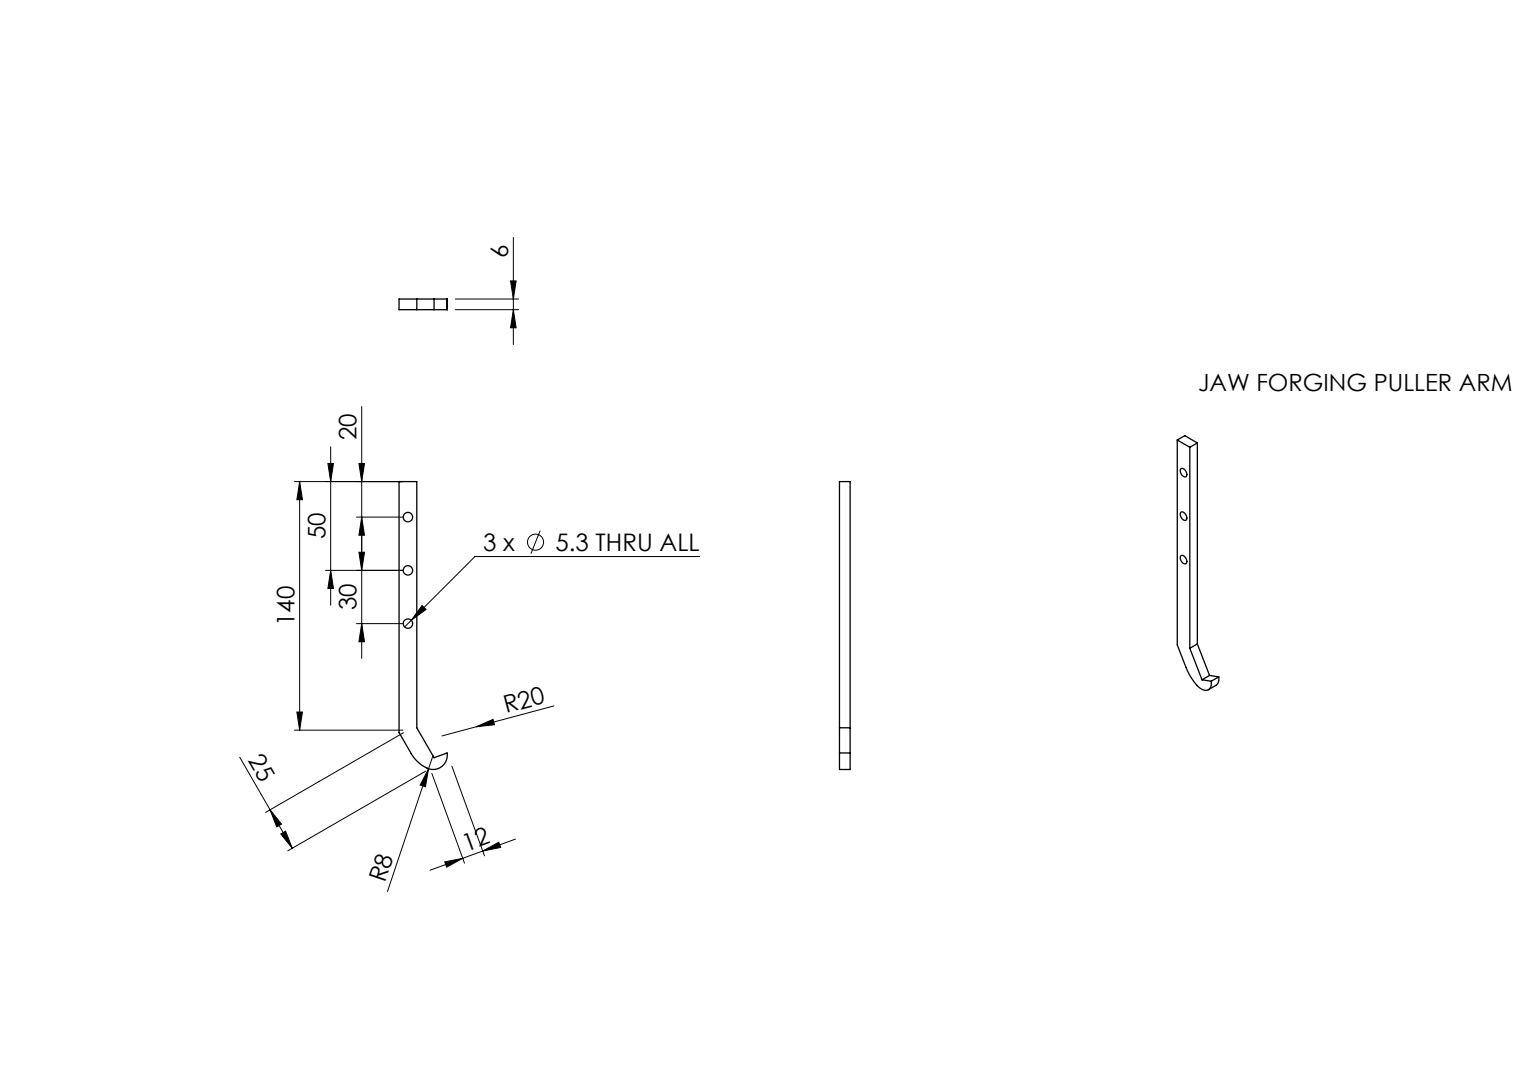
ISO-10303-21;
HEADER;
FILE_DESCRIPTION (('STEP AP214'),
    '1' );
FILE_NAME ('Jaw Forging Puller Arm.step',
    '2026-10-22T13:24:12',
    ( '' ),
    ( '' ),
    'SwSTEP 2.0',
    'SolidWorks 2026',
    '' );
FILE_SCHEMA (( 'AUTOMOTIVE_DESIGN' ));
ENDSEC;

DATA;
#1=DIRECTION ( 'NONE',  ( 1.000000000000000000, 0.000000000000000000, 0.000000000000000000 ) ) ;
#20=PRODUCT_DEFINITION_SHAPE ( 'NONE', 'NONE',  #1387 ) ;
#22=VECTOR ( 'NONE', #2319, 1000.000000000000000 ) ;
#55=EDGE_CURVE ( 'NONE', #2070, #608, #62, .T. ) ;
#59=CARTESIAN_POINT ( 'NONE',  ( -58.09974666316955449, -143.2580143298517328, -3.000000000000000000 ) ) ;
#62=CIRCLE ( 'NONE', #204, 20.00000000000000355 ) ;
#63=AXIS2_PLACEMENT_3D ( 'NONE', #554, #2133, #1693 ) ;
#75=EDGE_CURVE ( 'NONE', #120, #1771, #154, .T. ) ;
#76=CYLINDRICAL_SURFACE ( 'NONE', #302, 2.649999999999985700 ) ;
#78=LINE ( 'NONE', #2340, #2456 ) ;
#83=VERTEX_POINT ( 'NONE', #98 ) ;
#91=DIRECTION ( 'NONE',  ( -0.000000000000000000, -0.000000000000000000, 1.000000000000000000 ) ) ;
#93=VERTEX_POINT ( 'NONE', #2360 ) ;
#94=AXIS2_PLACEMENT_3D ( 'NONE', #273, #1403, #2068 ) ;
#98=CARTESIAN_POINT ( 'NONE',  ( -62.63076211353318712, -9.999999999999943157, 3.000000000000001332 ) ) ;
#109=CLOSED_SHELL ( 'NONE', ( #2797, #1837, #1415, #550, #392, #827, #441, #1532, #2192, #615, #2313, #2289, #2566, #2325, #660, #1443, #890 ) ) ;
#111=EDGE_CURVE ( 'NONE', #2201, #2834, #2628, .T. ) ;
#113=EDGE_CURVE ( 'NONE', #132, #2201, #803, .T. ) ;
#120=VERTEX_POINT ( 'NONE', #127 ) ;
#125=ORIENTED_EDGE ( 'NONE', *, *, #2038, .F. ) ;
#127=CARTESIAN_POINT ( 'NONE',  ( -37.91455138073065001, -142.8479302707733041, -3.000000000000000000 ) ) ;
#128=CARTESIAN_POINT ( 'NONE',  ( -62.63076211353317291, -39.99999999999994316, -3.000000000000005329 ) ) ;
#129=EDGE_CURVE ( 'NONE', #732, #608, #1011, .T. ) ;
#131=DIRECTION ( 'NONE',  ( -0.000000000000000000, -0.000000000000000000, 1.000000000000000000 ) ) ;
#132=VERTEX_POINT ( 'NONE', #1872 ) ;
#134=( NAMED_UNIT ( * ) PLANE_ANGLE_UNIT ( ) SI_UNIT ( $, .RADIAN. ) );
#143=CARTESIAN_POINT ( 'NONE',  ( -57.33076211353320417, -69.99999999999995737, 3.000000000000001332 ) ) ;
#152=EDGE_CURVE ( 'NONE', #1771, #732, #1431, .T. ) ;
#154=CIRCLE ( 'NONE', #1792, 8.000000000000000000 ) ;
#160=DIRECTION ( 'NONE',  ( 1.000000000000000000, 0.000000000000000000, 0.000000000000000000 ) ) ;
#167=VERTEX_POINT ( 'NONE', #2852 ) ;
#171=ORIENTED_EDGE ( 'NONE', *, *, #2056, .F. ) ;
#175=DIRECTION ( 'NONE',  ( 1.000000000000000000, 0.000000000000000000, 0.000000000000000000 ) ) ;
#177=ORIENTED_EDGE ( 'NONE', *, *, #2792, .T. ) ;
#190=LINE ( 'NONE', #904, #997 ) ;
#197=VECTOR ( 'NONE', #522, 1000.000000000000000 ) ;
#199=EDGE_CURVE ( 'NONE', #2240, #2529, #1039, .T. ) ;
#204=AXIS2_PLACEMENT_3D ( 'NONE', #900, #2724, #531 ) ;
#211=CARTESIAN_POINT ( 'NONE',  ( -59.98076211353318854, -69.99999999999995737, 3.000000000000000000 ) ) ;
#212=VECTOR ( 'NONE', #1969, 1000.000000000000000 ) ;
#214=LINE ( 'NONE', #690, #2553 ) ;
#219=EDGE_CURVE ( 'NONE', #1447, #1073, #1678, .T. ) ;
#223=DIRECTION ( 'NONE',  ( -1.000000000000000000, 0.000000000000000000, 0.000000000000000000 ) ) ;
#224=CARTESIAN_POINT ( 'NONE',  ( -59.98076211353319565, -9.999999999999943157, 3.000000000000000000 ) ) ;
#230=CARTESIAN_POINT ( 'NONE',  ( -64.98076211353318854, 10.00000000000005684, -3.000000000000000000 ) ) ;
#231=CARTESIAN_POINT ( 'NONE',  ( 0.000000000000000000, 0.000000000000000000, 0.000000000000000000 ) ) ;
#232=ORIENTED_EDGE ( 'NONE', *, *, #2574, .F. ) ;
#233=EDGE_CURVE ( 'NONE', #1447, #2315, #1733, .T. ) ;
#245=DIRECTION ( 'NONE',  ( 0.000000000000000000, 0.000000000000000000, 1.000000000000000000 ) ) ;
#247=ORIENTED_EDGE ( 'NONE', *, *, #2110, .T. ) ;
#249=CARTESIAN_POINT ( 'NONE',  ( -37.80724301738815285, -144.1538470861320604, -3.000000000000000000 ) ) ;
#252=CARTESIAN_POINT ( 'NONE',  ( -40.77923858748079766, -133.2580143298517044, -3.000000000000000000 ) ) ;
#254=VECTOR ( 'NONE', #2412, 1000.000000000000000 ) ;
#257=EDGE_CURVE ( 'NONE', #2834, #1447, #2641, .T. ) ;
#263=SURFACE_STYLE_USAGE ( .BOTH. , #928 ) ;
#266=( NAMED_UNIT ( * ) PLANE_ANGLE_UNIT ( ) SI_UNIT ( $, .RADIAN. ) );
#270=CARTESIAN_POINT ( 'NONE',  ( -49.19086283016151384, -146.9521719906813928, 3.000000000000000000 ) ) ;
#273=CARTESIAN_POINT ( 'NONE',  ( 0.000000000000000000, 0.000000000000000000, -3.000000000000000000 ) ) ;
#274=ORIENTED_EDGE ( 'NONE', *, *, #2038, .T. ) ;
#277=ORIENTED_EDGE ( 'NONE', *, *, #2792, .F. ) ;
#281=CARTESIAN_POINT ( 'NONE',  ( -59.98076211353318854, -69.99999999999995737, -3.000000000000005329 ) ) ;
#282=EDGE_CURVE ( 'NONE', #300, #2070, #409, .T. ) ;
#289=ORIENTED_EDGE ( 'NONE', *, *, #762, .F. ) ;
#295=VECTOR ( 'NONE', #821, 1000.000000000000000 ) ;
#300=VERTEX_POINT ( 'NONE', #2011 ) ;
#302=AXIS2_PLACEMENT_3D ( 'NONE', #1642, #1876, #2515 ) ;
#305=EDGE_LOOP ( 'NONE', ( #581, #1424, #2061, #2597 ) ) ;
#308=CARTESIAN_POINT ( 'NONE',  ( -55.65063509461099045, -127.4999999999999432, 3.000000000000000000 ) ) ;
#311=CARTESIAN_POINT ( 'NONE',  ( -62.63076211353317291, -69.99999999999995737, 3.000000000000000000 ) ) ;
#322=DIRECTION ( 'NONE',  ( 0.000000000000000000, -0.000000000000000000, 1.000000000000000000 ) ) ;
#333=CARTESIAN_POINT ( 'NONE',  ( -59.98076211353318854, -69.99999999999995737, 3.000000000000001332 ) ) ;
#334=ORIENTED_EDGE ( 'NONE', *, *, #1164, .F. ) ;
#336=AXIS2_PLACEMENT_3D ( 'NONE', #211, #2698, #2453 ) ;
#352=DIRECTION ( 'NONE',  ( 0.8660254037844379305, 0.5000000000000014433, -0.000000000000000000 ) ) ;
#356=DIRECTION ( 'NONE',  ( 1.000000000000000000, 0.000000000000000000, 0.000000000000000000 ) ) ;
#374=VECTOR ( 'NONE', #2202, 1000.000000000000000 ) ;
#378=ORIENTED_EDGE ( 'NONE', *, *, #113, .F. ) ;
#379=DIRECTION ( 'NONE',  ( -0.000000000000000000, -0.000000000000000000, 1.000000000000000000 ) ) ;
#384=CARTESIAN_POINT ( 'NONE',  ( -62.63076211353317291, -69.99999999999995737, 3.000000000000001332 ) ) ;
#387=CARTESIAN_POINT ( 'NONE',  ( -59.98076211353318854, -69.99999999999995737, 3.000000000000001332 ) ) ;
#388=VECTOR ( 'NONE', #1937, 1000.000000000000000 ) ;
#390=CARTESIAN_POINT ( 'NONE',  ( -54.98076211353318143, -128.6602540378443393, 3.000000000000000000 ) ) ;
#392=ADVANCED_FACE ( 'NONE', ( #2249 ), #1339, .T. ) ;
#401=CARTESIAN_POINT ( 'NONE',  ( -57.33076211353320417, -39.99999999999994316, -3.000000000000005329 ) ) ;
#409=LINE ( 'NONE', #626, #254 ) ;
#413=DIRECTION ( 'NONE',  ( -0.000000000000000000, -0.000000000000000000, 1.000000000000000000 ) ) ;
#416=AXIS2_PLACEMENT_3D ( 'NONE', #1762, #636, #1319 ) ;
#417=CARTESIAN_POINT ( 'NONE',  ( -45.80724301738815285, -144.1538470861320604, 3.000000000000000000 ) ) ;
#419=VECTOR ( 'NONE', #558, 1000.000000000000000 ) ;
#432=EDGE_LOOP ( 'NONE', ( #247, #171, #2273, #2867 ) ) ;
#434=CIRCLE ( 'NONE', #2909, 8.000000000000000000 ) ;
#436=VECTOR ( 'NONE', #2543, 1000.000000000000000 ) ;
#440=DIRECTION ( 'NONE',  ( -0.000000000000000000, -0.000000000000000000, 1.000000000000000000 ) ) ;
#441=ADVANCED_FACE ( 'NONE', ( #2720 ), #2522, .T. ) ;
#454=ORIENTED_EDGE ( 'NONE', *, *, #762, .T. ) ;
#466=COLOUR_RGB ( '',0.8941176470588234615, 0.8941176470588234615, 0.8941176470588234615 ) ;
#469=VECTOR ( 'NONE', #91, 1000.000000000000000 ) ;
#473=CYLINDRICAL_SURFACE ( 'NONE', #1427, 2.649999999999985700 ) ;
#478=UNCERTAINTY_MEASURE_WITH_UNIT (LENGTH_MEASURE( 1.000000000000000082E-05 ), #1953, 'distance_accuracy_value', 'NONE');
#487=ORIENTED_EDGE ( 'NONE', *, *, #685, .T. ) ;
#489=DIRECTION ( 'NONE',  ( -0.000000000000000000, -0.000000000000000000, 1.000000000000000000 ) ) ;
#495=EDGE_CURVE ( 'NONE', #1073, #120, #1819, .T. ) ;
#501=CARTESIAN_POINT ( 'NONE',  ( -62.63076211353318712, -9.999999999999943157, 3.000000000000000000 ) ) ;
#503=CARTESIAN_POINT ( 'NONE',  ( -57.33076211353320417, -69.99999999999995737, -3.000000000000005329 ) ) ;
#506=CARTESIAN_POINT ( 'NONE',  ( -62.63076211353317291, -39.99999999999994316, 3.000000000000000000 ) ) ;
#510=AXIS2_PLACEMENT_3D ( 'NONE', #2538, #1421, #1142 ) ;
#511=CARTESIAN_POINT ( 'NONE',  ( 0.000000000000000000, 0.000000000000000000, 3.000000000000000000 ) ) ;
#514=EDGE_CURVE ( 'NONE', #1931, #1630, #755, .T. ) ;
#522=DIRECTION ( 'NONE',  ( -0.000000000000000000, -0.000000000000000000, 1.000000000000000000 ) ) ;
#531=DIRECTION ( 'NONE',  ( -1.000000000000000000, 0.000000000000000000, 0.000000000000000000 ) ) ;
#536=CARTESIAN_POINT ( 'NONE',  ( -64.98076211353318854, 10.00000000000005684, 3.000000000000000000 ) ) ;
#546=DIRECTION ( 'NONE',  ( -0.000000000000000000, -0.000000000000000000, 1.000000000000000000 ) ) ;
#550=ADVANCED_FACE ( 'NONE', ( #589 ), #2548, .T. ) ;
#554=CARTESIAN_POINT ( 'NONE',  ( -45.80724301738815285, -144.1538470861320604, -3.000000000000000000 ) ) ;
#557=AXIS2_PLACEMENT_3D ( 'NONE', #1093, #1120, #664 ) ;
#558=DIRECTION ( 'NONE',  ( -0.000000000000000000, -0.000000000000000000, 1.000000000000000000 ) ) ;
#560=ORIENTED_EDGE ( 'NONE', *, *, #1193, .F. ) ;
#561=PLANE ( 'NONE',  #1135 ) ;
#563=ORIENTED_EDGE ( 'NONE', *, *, #2156, .F. ) ;
#564=AXIS2_PLACEMENT_3D ( 'NONE', #270, #2042, #727 ) ;
#575=ORIENTED_EDGE ( 'NONE', *, *, #2314, .T. ) ;
#578=EDGE_LOOP ( 'NONE', ( #232, #588 ) ) ;
#581=ORIENTED_EDGE ( 'NONE', *, *, #782, .F. ) ;
#583=EDGE_CURVE ( 'NONE', #1771, #167, #812, .T. ) ;
#586=LINE ( 'NONE', #1489, #295 ) ;
#588=ORIENTED_EDGE ( 'NONE', *, *, #1702, .F. ) ;
#589=FACE_OUTER_BOUND ( 'NONE', #1154, .T. ) ;
#591=CARTESIAN_POINT ( 'NONE',  ( -40.77923858748079766, -133.2580143298517044, 3.000000000000000000 ) ) ;
#606=EDGE_LOOP ( 'NONE', ( #2745, #2300, #1536, #1449, #625, #2303, #454, #2564, #695 ) ) ;
#608=VERTEX_POINT ( 'NONE', #2604 ) ;
#615=ADVANCED_FACE ( 'NONE', ( #1270 ), #561, .F. ) ;
#623=DIRECTION ( 'NONE',  ( -1.000000000000000000, 0.000000000000000000, 0.000000000000000000 ) ) ;
#625=ORIENTED_EDGE ( 'NONE', *, *, #1622, .F. ) ;
#626=CARTESIAN_POINT ( 'NONE',  ( -64.31088913245535821, -132.4999999999999432, 3.000000000000000000 ) ) ;
#634=EDGE_CURVE ( 'NONE', #2529, #2240, #2044, .T. ) ;
#636=DIRECTION ( 'NONE',  ( -0.000000000000000000, -0.000000000000000000, 1.000000000000000000 ) ) ;
#645=DIRECTION ( 'NONE',  ( -0.000000000000000000, -0.000000000000000000, 1.000000000000000000 ) ) ;
#653=ORIENTED_EDGE ( 'NONE', *, *, #752, .F. ) ;
#660=ADVANCED_FACE ( 'NONE', ( #798 ), #1966, .F. ) ;
#664=DIRECTION ( 'NONE',  ( -1.000000000000000000, 3.469446951953614189E-15, 0.000000000000000000 ) ) ;
#682=FACE_OUTER_BOUND ( 'NONE', #606, .T. ) ;
#685=EDGE_CURVE ( 'NONE', #167, #1073, #434, .T. ) ;
#688=CARTESIAN_POINT ( 'NONE',  ( -64.98076211353318854, 10.00000000000005684, 3.000000000000000000 ) ) ;
#690=CARTESIAN_POINT ( 'NONE',  ( -49.19086283016151384, -146.9521719906813928, -3.000000000000000000 ) ) ;
#695=ORIENTED_EDGE ( 'NONE', *, *, #1164, .T. ) ;
#707=PLANE ( 'NONE',  #2476 ) ;
#712=CIRCLE ( 'NONE', #1563, 2.649999999999985700 ) ;
#716=FACE_BOUND ( 'NONE', #813, .T. ) ;
#717=EDGE_LOOP ( 'NONE', ( #289, #2875, #2214, #2681 ) ) ;
#719=FACE_OUTER_BOUND ( 'NONE', #1079, .T. ) ;
#721=LINE ( 'NONE', #688, #436 ) ;
#722=FACE_OUTER_BOUND ( 'NONE', #717, .T. ) ;
#727=DIRECTION ( 'NONE',  ( -0.9396926207859063185, -0.3420201433256743195, 0.000000000000000000 ) ) ;
#728=FACE_BOUND ( 'NONE', #2290, .T. ) ;
#732=VERTEX_POINT ( 'NONE', #2497 ) ;
#736=VECTOR ( 'NONE', #1465, 1000.000000000000000 ) ;
#741=VERTEX_POINT ( 'NONE', #1537 ) ;
#742=DIRECTION ( 'NONE',  ( 1.000000000000000000, 0.000000000000000000, 0.000000000000000000 ) ) ;
#748=CARTESIAN_POINT ( 'NONE',  ( -62.63076211353317291, -69.99999999999995737, -3.000000000000005329 ) ) ;
#752=EDGE_CURVE ( 'NONE', #2529, #1384, #190, .T. ) ;
#755=CIRCLE ( 'NONE', #2422, 2.649999999999985700 ) ;
#760=DIRECTION ( 'NONE',  ( -1.000000000000000000, 0.000000000000000000, 0.000000000000000000 ) ) ;
#762=EDGE_CURVE ( 'NONE', #1742, #1508, #2230, .T. ) ;
#767=ORIENTED_EDGE ( 'NONE', *, *, #75, .F. ) ;
#770=DIRECTION ( 'NONE',  ( -0.000000000000000000, -0.000000000000000000, 1.000000000000000000 ) ) ;
#777=CARTESIAN_POINT ( 'NONE',  ( -37.80724301738815285, -144.1538470861320604, 3.000000000000000000 ) ) ;
#782=EDGE_CURVE ( 'NONE', #814, #969, #712, .T. ) ;
#788=CIRCLE ( 'NONE', #1596, 2.649999999999985700 ) ;
#792=AXIS2_PLACEMENT_3D ( 'NONE', #224, #2741, #1523 ) ;
#794=FACE_OUTER_BOUND ( 'NONE', #1190, .T. ) ;
#795=STYLED_ITEM('',(#2956),#1538);
#797=ORIENTED_EDGE ( 'NONE', *, *, #583, .F. ) ;
#798=FACE_OUTER_BOUND ( 'NONE', #1917, .T. ) ;
#800=ORIENTED_EDGE ( 'NONE', *, *, #1284, .T. ) ;
#803=LINE ( 'NONE', #1707, #1373 ) ;
#812=LINE ( 'NONE', #777, #2141 ) ;
#813=EDGE_LOOP ( 'NONE', ( #800, #1999 ) ) ;
#814=VERTEX_POINT ( 'NONE', #748 ) ;
#821=DIRECTION ( 'NONE',  ( 0.5000000000000013323, -0.8660254037844379305, 0.000000000000000000 ) ) ;
#827=ADVANCED_FACE ( 'NONE', ( #2062 ), #707, .T. ) ;
#832=ORIENTED_EDGE ( 'NONE', *, *, #872, .F. ) ;
#837=ORIENTED_EDGE ( 'NONE', *, *, #199, .T. ) ;
#843=CARTESIAN_POINT ( 'NONE',  ( -62.63076211353317291, -39.99999999999994316, 3.000000000000001332 ) ) ;
#844=ORIENTED_EDGE ( 'NONE', *, *, #514, .T. ) ;
#851=AXIS2_PLACEMENT_3D ( 'NONE', #1018, #379, #1728 ) ;
#854=VECTOR ( 'NONE', #546, 1000.000000000000000 ) ;
#857=LINE ( 'NONE', #1534, #1783 ) ;
#858=ORIENTED_EDGE ( 'NONE', *, *, #1284, .F. ) ;
#860=CYLINDRICAL_SURFACE ( 'NONE', #336, 2.649999999999985700 ) ;
#866=SHAPE_DEFINITION_REPRESENTATION ( #20, #1396 ) ;
#872=EDGE_CURVE ( 'NONE', #2834, #93, #916, .T. ) ;
#887=PRODUCT_DEFINITION_CONTEXT ( 'detailed design', #2350, 'design' ) ;
#890=ADVANCED_FACE ( 'NONE', ( #2291 ), #76, .F. ) ;
#900=CARTESIAN_POINT ( 'NONE',  ( -40.77923858748079766, -133.2580143298517044, 3.000000000000000000 ) ) ;
#904=CARTESIAN_POINT ( 'NONE',  ( -57.33076211353321128, -9.999999999999943157, 3.000000000000000000 ) ) ;
#908=VERTEX_POINT ( 'NONE', #59 ) ;
#909=DIRECTION ( 'NONE',  ( 1.000000000000000000, 1.486905836551548586E-16, -0.000000000000000000 ) ) ;
#916=LINE ( 'NONE', #1395, #22 ) ;
#921=ORIENTED_EDGE ( 'NONE', *, *, #1009, .T. ) ;
#928=SURFACE_SIDE_STYLE ('',( #1344 ) ) ;
#941=AXIS2_PLACEMENT_3D ( 'NONE', #536, #2097, #322 ) ;
#944=CARTESIAN_POINT ( 'NONE',  ( -59.98076211353319565, -9.999999999999943157, 3.000000000000000000 ) ) ;
#954=ORIENTED_EDGE ( 'NONE', *, *, #2516, .F. ) ;
#956=FACE_OUTER_BOUND ( 'NONE', #2363, .T. ) ;
#959=DIRECTION ( 'NONE',  ( -0.000000000000000000, -0.000000000000000000, 1.000000000000000000 ) ) ;
#962=LINE ( 'NONE', #1832, #2751 ) ;
#964=EDGE_CURVE ( 'NONE', #132, #300, #721, .T. ) ;
#968=DIRECTION ( 'NONE',  ( 0.000000000000000000, 0.000000000000000000, -1.000000000000000000 ) ) ;
#969=VERTEX_POINT ( 'NONE', #503 ) ;
#986=( GEOMETRIC_REPRESENTATION_CONTEXT ( 3 ) GLOBAL_UNCERTAINTY_ASSIGNED_CONTEXT ( ( #478 ) ) GLOBAL_UNIT_ASSIGNED_CONTEXT ( ( #1953, #134, #1510 ) ) REPRESENTATION_CONTEXT ( 'NONE', 'WORKASPACE' ) );
#995=ORIENTED_EDGE ( 'NONE', *, *, #583, .T. ) ;
#997=VECTOR ( 'NONE', #2713, 1000.000000000000000 ) ;
#1009=EDGE_CURVE ( 'NONE', #969, #1547, #2586, .T. ) ;
#1011=LINE ( 'NONE', #1668, #2903 ) ;
#1013=CARTESIAN_POINT ( 'NONE',  ( -64.98076211353316012, -131.3397459621555754, 3.000000000000000000 ) ) ;
#1014=ORIENTED_EDGE ( 'NONE', *, *, #634, .T. ) ;
#1018=CARTESIAN_POINT ( 'NONE',  ( -59.98076211353319565, -9.999999999999943157, -3.000000000000005329 ) ) ;
#1020=AXIS2_PLACEMENT_3D ( 'NONE', #1980, #2677, #1529 ) ;
#1028=PRODUCT_DEFINITION_FORMATION_WITH_SPECIFIED_SOURCE ( 'ANY', '', #1535, .NOT_KNOWN. ) ;
#1039=CIRCLE ( 'NONE', #1230, 2.649999999999985700 ) ;
#1058=VERTEX_POINT ( 'NONE', #843 ) ;
#1062=ORIENTED_EDGE ( 'NONE', *, *, #1866, .T. ) ;
#1073=VERTEX_POINT ( 'NONE', #2213 ) ;
#1077=MECHANICAL_DESIGN_GEOMETRIC_PRESENTATION_REPRESENTATION('',(#795),#1983);
#1079=EDGE_LOOP ( 'NONE', ( #2132, #1062, #575, #653 ) ) ;
#1080=EDGE_LOOP ( 'NONE', ( #1185, #1761, #1889, #1111 ) ) ;
#1082=AXIS2_PLACEMENT_3D ( 'NONE', #1112, #909, #2264 ) ;
#1091=ORIENTED_EDGE ( 'NONE', *, *, #55, .T. ) ;
#1093=CARTESIAN_POINT ( 'NONE',  ( -45.80724301738815285, -144.1538470861320604, 3.000000000000000000 ) ) ;
#1096=DIRECTION ( 'NONE',  ( 0.9396926207859063185, 0.3420201433256743750, 0.000000000000000000 ) ) ;
#1105=ORIENTED_EDGE ( 'NONE', *, *, #282, .T. ) ;
#1111=ORIENTED_EDGE ( 'NONE', *, *, #872, .T. ) ;
#1112=CARTESIAN_POINT ( 'NONE',  ( -54.98076211353320275, 10.00000000000005684, 3.000000000000000000 ) ) ;
#1120=DIRECTION ( 'NONE',  ( -0.000000000000000000, -0.000000000000000000, 1.000000000000000000 ) ) ;
#1127=DIRECTION ( 'NONE',  ( 1.000000000000000000, 0.000000000000000000, 0.000000000000000000 ) ) ;
#1128=EDGE_LOOP ( 'NONE', ( #1388, #2021, #1429, #2033 ) ) ;
#1134=CARTESIAN_POINT ( 'NONE',  ( -59.98076211353318854, -69.99999999999995737, -3.000000000000005329 ) ) ;
#1135=AXIS2_PLACEMENT_3D ( 'NONE', #2635, #352, #2407 ) ;
#1142=DIRECTION ( 'NONE',  ( 1.000000000000000000, 0.000000000000000000, 0.000000000000000000 ) ) ;
#1146=ORIENTED_EDGE ( 'NONE', *, *, #282, .F. ) ;
#1154=EDGE_LOOP ( 'NONE', ( #2301, #995, #1242, #2705 ) ) ;
#1164=EDGE_CURVE ( 'NONE', #93, #2315, #2008, .T. ) ;
#1167=CARTESIAN_POINT ( 'NONE',  ( -37.91455138073065001, -142.8479302707733041, 3.000000000000000000 ) ) ;
#1185=ORIENTED_EDGE ( 'NONE', *, *, #2682, .F. ) ;
#1189=CARTESIAN_POINT ( 'NONE',  ( -62.63076211353318712, -9.999999999999943157, -3.000000000000005329 ) ) ;
#1190=EDGE_LOOP ( 'NONE', ( #1875, #1724, #1194, #277 ) ) ;
#1193=EDGE_CURVE ( 'NONE', #1630, #1931, #2463, .T. ) ;
#1194=ORIENTED_EDGE ( 'NONE', *, *, #1702, .T. ) ;
#1223=DIRECTION ( 'NONE',  ( 1.000000000000000000, 0.000000000000000000, 0.000000000000000000 ) ) ;
#1225=( NAMED_UNIT ( * ) SI_UNIT ( $, .STERADIAN. ) SOLID_ANGLE_UNIT ( ) );
#1230=AXIS2_PLACEMENT_3D ( 'NONE', #2104, #770, #742 ) ;
#1241=CARTESIAN_POINT ( 'NONE',  ( -59.98076211353319565, -9.999999999999943157, 3.000000000000001332 ) ) ;
#1242=ORIENTED_EDGE ( 'NONE', *, *, #1342, .F. ) ;
#1253=CARTESIAN_POINT ( 'NONE',  ( -59.98076211353318854, -39.99999999999994316, -3.000000000000005329 ) ) ;
#1263=AXIS2_PLACEMENT_3D ( 'NONE', #281, #1399, #1662 ) ;
#1266=EDGE_CURVE ( 'NONE', #1931, #1058, #1414, .T. ) ;
#1270=FACE_OUTER_BOUND ( 'NONE', #2023, .T. ) ;
#1272=FILL_AREA_STYLE_COLOUR ( '', #466 ) ;
#1274=VECTOR ( 'NONE', #1301, 1000.000000000000000 ) ;
#1278=FACE_OUTER_BOUND ( 'NONE', #432, .T. ) ;
#1283=DIRECTION ( 'NONE',  ( 0.000000000000000000, 0.000000000000000000, 1.000000000000000000 ) ) ;
#1284=EDGE_CURVE ( 'NONE', #969, #814, #2127, .T. ) ;
#1291=LINE ( 'NONE', #2238, #2119 ) ;
#1301=DIRECTION ( 'NONE',  ( 0.9396926207859063185, 0.3420201433256743750, 0.000000000000000000 ) ) ;
#1306=EDGE_LOOP ( 'NONE', ( #2804, #1970 ) ) ;
#1309=DIRECTION ( 'NONE',  ( 1.000000000000000000, 0.000000000000000000, 0.000000000000000000 ) ) ;
#1319=DIRECTION ( 'NONE',  ( 1.000000000000000000, 0.000000000000000000, 0.000000000000000000 ) ) ;
#1335=DIRECTION ( 'NONE',  ( -1.000000000000000000, 0.000000000000000000, 0.000000000000000000 ) ) ;
#1339=PLANE ( 'NONE',  #564 ) ;
#1341=EDGE_LOOP ( 'NONE', ( #2912, #1696, #1648, #1407 ) ) ;
#1342=EDGE_CURVE ( 'NONE', #608, #167, #1649, .T. ) ;
#1344=SURFACE_STYLE_FILL_AREA ( #2185 ) ;
#1351=ORIENTED_EDGE ( 'NONE', *, *, #233, .T. ) ;
#1355=FACE_BOUND ( 'NONE', #1525, .T. ) ;
#1364=DIRECTION ( 'NONE',  ( 1.000000000000000000, 0.000000000000000000, 0.000000000000000000 ) ) ;
#1373=VECTOR ( 'NONE', #356, 1000.000000000000000 ) ;
#1379=VECTOR ( 'NONE', #2894, 1000.000000000000000 ) ;
#1384=VERTEX_POINT ( 'NONE', #1539 ) ;
#1387=PRODUCT_DEFINITION ( 'UNKNOWN', '', #1028, #887 ) ;
#1388=ORIENTED_EDGE ( 'NONE', *, *, #1866, .F. ) ;
#1395=CARTESIAN_POINT ( 'NONE',  ( -54.98076211353318143, -128.6602540378443393, 3.000000000000000000 ) ) ;
#1396=SHAPE_REPRESENTATION ( 'Jaw Forging Puller Arm', ( #2652 ), #986 ) ;
#1397=CARTESIAN_POINT ( 'NONE',  ( -54.98076211353320275, 10.00000000000005684, -3.000000000000000000 ) ) ;
#1399=DIRECTION ( 'NONE',  ( -0.000000000000000000, -0.000000000000000000, 1.000000000000000000 ) ) ;
#1403=DIRECTION ( 'NONE',  ( 0.000000000000000000, 0.000000000000000000, -1.000000000000000000 ) ) ;
#1405=ORIENTED_EDGE ( 'NONE', *, *, #233, .F. ) ;
#1407=ORIENTED_EDGE ( 'NONE', *, *, #2915, .F. ) ;
#1414=LINE ( 'NONE', #506, #469 ) ;
#1415=ADVANCED_FACE ( 'NONE', ( #2730 ), #860, .F. ) ;
#1417=EDGE_LOOP ( 'NONE', ( #797, #767, #2780, #1466 ) ) ;
#1421=DIRECTION ( 'NONE',  ( -0.000000000000000000, -0.000000000000000000, 1.000000000000000000 ) ) ;
#1424=ORIENTED_EDGE ( 'NONE', *, *, #1493, .T. ) ;
#1427=AXIS2_PLACEMENT_3D ( 'NONE', #944, #489, #2572 ) ;
#1428=EDGE_CURVE ( 'NONE', #732, #908, #1926, .T. ) ;
#1429=ORIENTED_EDGE ( 'NONE', *, *, #752, .T. ) ;
#1430=DIRECTION ( 'NONE',  ( -0.5000000000000013323, 0.8660254037844378194, 0.000000000000000000 ) ) ;
#1431=CIRCLE ( 'NONE', #63, 8.000000000000000000 ) ;
#1443=ADVANCED_FACE ( 'NONE', ( #1815 ), #2244, .F. ) ;
#1447=VERTEX_POINT ( 'NONE', #2438 ) ;
#1449=ORIENTED_EDGE ( 'NONE', *, *, #1428, .T. ) ;
#1450=DIRECTION ( 'NONE',  ( 0.000000000000000000, 0.000000000000000000, -1.000000000000000000 ) ) ;
#1465=DIRECTION ( 'NONE',  ( -0.000000000000000000, -0.000000000000000000, -1.000000000000000000 ) ) ;
#1466=ORIENTED_EDGE ( 'NONE', *, *, #685, .F. ) ;
#1472=EDGE_CURVE ( 'NONE', #132, #1742, #962, .T. ) ;
#1474=CARTESIAN_POINT ( 'NONE',  ( -54.98076211353320275, 10.00000000000005684, 3.000000000000000000 ) ) ;
#1478=LINE ( 'NONE', #2633, #419 ) ;
#1480=DIRECTION ( 'NONE',  ( 1.000000000000000000, 0.000000000000000000, 0.000000000000000000 ) ) ;
#1482=APPLICATION_CONTEXT ( 'automotive_design' ) ;
#1489=CARTESIAN_POINT ( 'NONE',  ( -64.31088913245535821, -132.4999999999999432, -3.000000000000000000 ) ) ;
#1493=EDGE_CURVE ( 'NONE', #814, #2489, #2758, .T. ) ;
#1496=LINE ( 'NONE', #1816, #374 ) ;
#1508=VERTEX_POINT ( 'NONE', #1397 ) ;
#1510=( NAMED_UNIT ( * ) SI_UNIT ( $, .STERADIAN. ) SOLID_ANGLE_UNIT ( ) );
#1518=CARTESIAN_POINT ( 'NONE',  ( -59.98076211353318854, -39.99999999999994316, 3.000000000000001332 ) ) ;
#1523=DIRECTION ( 'NONE',  ( 1.000000000000000000, 0.000000000000000000, 0.000000000000000000 ) ) ;
#1525=EDGE_LOOP ( 'NONE', ( #2931, #844 ) ) ;
#1529=DIRECTION ( 'NONE',  ( -1.486905836551548586E-16, 1.000000000000000000, 0.000000000000000000 ) ) ;
#1532=ADVANCED_FACE ( 'NONE', ( #722 ), #1628, .T. ) ;
#1534=CARTESIAN_POINT ( 'NONE',  ( -58.09974666316955449, -143.2580143298517328, 3.000000000000000000 ) ) ;
#1535=PRODUCT ( 'Jaw Forging Puller Arm', 'Jaw Forging Puller Arm', '', ( #2221 ) ) ;
#1536=ORIENTED_EDGE ( 'NONE', *, *, #152, .T. ) ;
#1537=CARTESIAN_POINT ( 'NONE',  ( -64.98076211353316012, -131.3397459621555754, -3.000000000000000000 ) ) ;
#1538=MANIFOLD_SOLID_BREP ( 'M5 Clearance Hole1', #109 ) ;
#1539=CARTESIAN_POINT ( 'NONE',  ( -57.33076211353321128, -9.999999999999943157, 3.000000000000001332 ) ) ;
#1547=VERTEX_POINT ( 'NONE', #143 ) ;
#1563=AXIS2_PLACEMENT_3D ( 'NONE', #1134, #2017, #1 ) ;
#1574=CYLINDRICAL_SURFACE ( 'NONE', #2122, 8.000000000000000000 ) ;
#1596=AXIS2_PLACEMENT_3D ( 'NONE', #1241, #2150, #160 ) ;
#1599=( LENGTH_UNIT ( ) NAMED_UNIT ( * ) SI_UNIT ( .MILLI., .METRE. ) );
#1619=PLANE ( 'NONE',  #1880 ) ;
#1622=EDGE_CURVE ( 'NONE', #741, #908, #586, .T. ) ;
#1627=DIRECTION ( 'NONE',  ( 0.8660254037844379305, 0.5000000000000014433, -0.000000000000000000 ) ) ;
#1628=PLANE ( 'NONE',  #941 ) ;
#1630=VERTEX_POINT ( 'NONE', #401 ) ;
#1634=DIRECTION ( 'NONE',  ( -0.000000000000000000, -0.000000000000000000, 1.000000000000000000 ) ) ;
#1636=FACE_BOUND ( 'NONE', #578, .T. ) ;
#1639=ORIENTED_EDGE ( 'NONE', *, *, #2915, .T. ) ;
#1642=CARTESIAN_POINT ( 'NONE',  ( -59.98076211353318854, -39.99999999999994316, 3.000000000000000000 ) ) ;
#1648=ORIENTED_EDGE ( 'NONE', *, *, #55, .F. ) ;
#1649=CIRCLE ( 'NONE', #557, 8.000000000000000000 ) ;
#1662=DIRECTION ( 'NONE',  ( 1.000000000000000000, 0.000000000000000000, 0.000000000000000000 ) ) ;
#1668=CARTESIAN_POINT ( 'NONE',  ( -49.15924597065973956, -151.4177355903189550, 3.000000000000000000 ) ) ;
#1678=LINE ( 'NONE', #2430, #1274 ) ;
#1685=DIRECTION ( 'NONE',  ( 0.000000000000000000, 0.000000000000000000, 1.000000000000000000 ) ) ;
#1691=STYLED_ITEM ( 'NONE', ( #2753 ), #2288 ) ;
#1693=DIRECTION ( 'NONE',  ( -1.000000000000000000, 0.000000000000000000, 0.000000000000000000 ) ) ;
#1696=ORIENTED_EDGE ( 'NONE', *, *, #129, .T. ) ;
#1700=CARTESIAN_POINT ( 'NONE',  ( -45.80724301738815285, -144.1538470861320604, 3.000000000000000000 ) ) ;
#1702=EDGE_CURVE ( 'NONE', #1058, #2820, #2710, .T. ) ;
#1707=CARTESIAN_POINT ( 'NONE',  ( -64.98076211353318854, 10.00000000000005684, 3.000000000000000000 ) ) ;
#1710=ORIENTED_EDGE ( 'NONE', *, *, #257, .F. ) ;
#1724=ORIENTED_EDGE ( 'NONE', *, *, #1266, .T. ) ;
#1728=DIRECTION ( 'NONE',  ( 1.000000000000000000, 0.000000000000000000, 0.000000000000000000 ) ) ;
#1732=EDGE_LOOP ( 'NONE', ( #334, #832, #1855, #1351 ) ) ;
#1733=LINE ( 'NONE', #1750, #1379 ) ;
#1742=VERTEX_POINT ( 'NONE', #230 ) ;
#1746=AXIS2_PLACEMENT_3D ( 'NONE', #1700, #1283, #175 ) ;
#1748=CYLINDRICAL_SURFACE ( 'NONE', #1971, 20.00000000000000355 ) ;
#1750=CARTESIAN_POINT ( 'NONE',  ( -45.24838417255416800, -145.5172271100825299, 3.000000000000000000 ) ) ;
#1755=DIRECTION ( 'NONE',  ( 1.000000000000000000, 0.000000000000000000, 0.000000000000000000 ) ) ;
#1761=ORIENTED_EDGE ( 'NONE', *, *, #2514, .F. ) ;
#1762=CARTESIAN_POINT ( 'NONE',  ( -59.98076211353318854, -39.99999999999994316, 3.000000000000001332 ) ) ;
#1766=( NAMED_UNIT ( * ) PLANE_ANGLE_UNIT ( ) SI_UNIT ( $, .RADIAN. ) );
#1771=VERTEX_POINT ( 'NONE', #249 ) ;
#1772=CARTESIAN_POINT ( 'NONE',  ( -64.98076211353318854, 10.00000000000005684, -3.000000000000000000 ) ) ;
#1783=VECTOR ( 'NONE', #2228, 1000.000000000000000 ) ;
#1790=CARTESIAN_POINT ( 'NONE',  ( -59.98076211353318854, -39.99999999999994316, -3.000000000000005329 ) ) ;
#1792=AXIS2_PLACEMENT_3D ( 'NONE', #2611, #1450, #760 ) ;
#1815=FACE_OUTER_BOUND ( 'NONE', #1128, .T. ) ;
#1816=CARTESIAN_POINT ( 'NONE',  ( -54.98076211353320275, 10.00000000000005684, 3.000000000000000000 ) ) ;
#1819=LINE ( 'NONE', #1167, #388 ) ;
#1822=AXIS2_PLACEMENT_3D ( 'NONE', #333, #2870, #1223 ) ;
#1832=CARTESIAN_POINT ( 'NONE',  ( -64.98076211353318854, 10.00000000000005684, 3.000000000000000000 ) ) ;
#1835=AXIS2_PLACEMENT_3D ( 'NONE', #1518, #413, #1755 ) ;
#1837=ADVANCED_FACE ( 'NONE', ( #719 ), #473, .F. ) ;
#1855=ORIENTED_EDGE ( 'NONE', *, *, #257, .T. ) ;
#1857=CARTESIAN_POINT ( 'NONE',  ( -54.98076211353320275, 10.00000000000005684, 3.000000000000000000 ) ) ;
#1866=EDGE_CURVE ( 'NONE', #2240, #83, #2737, .T. ) ;
#1869=CARTESIAN_POINT ( 'NONE',  ( -45.24838417255416800, -145.5172271100825299, -3.000000000000000000 ) ) ;
#1872=CARTESIAN_POINT ( 'NONE',  ( -64.98076211353318854, 10.00000000000005684, 3.000000000000000000 ) ) ;
#1875=ORIENTED_EDGE ( 'NONE', *, *, #514, .F. ) ;
#1876=DIRECTION ( 'NONE',  ( -0.000000000000000000, -0.000000000000000000, 1.000000000000000000 ) ) ;
#1880=AXIS2_PLACEMENT_3D ( 'NONE', #511, #968, #2525 ) ;
#1889=ORIENTED_EDGE ( 'NONE', *, *, #111, .T. ) ;
#1893=CARTESIAN_POINT ( 'NONE',  ( -57.33076211353320417, -69.99999999999995737, 3.000000000000000000 ) ) ;
#1916=CYLINDRICAL_SURFACE ( 'NONE', #2172, 2.649999999999985700 ) ;
#1917=EDGE_LOOP ( 'NONE', ( #2128, #858, #921, #274 ) ) ;
#1924=( GEOMETRIC_REPRESENTATION_CONTEXT ( 3 ) GLOBAL_UNCERTAINTY_ASSIGNED_CONTEXT ( ( #2740 ) ) GLOBAL_UNIT_ASSIGNED_CONTEXT ( ( #2445, #1766, #2431 ) ) REPRESENTATION_CONTEXT ( 'NONE', 'WORKASPACE' ) );
#1926=CIRCLE ( 'NONE', #1981, 20.00000000000000355 ) ;
#1927=DIRECTION ( 'NONE',  ( -0.000000000000000000, -0.000000000000000000, 1.000000000000000000 ) ) ;
#1929=SHAPE_REPRESENTATION_RELATIONSHIP ( 'NONE' , 'NONE' ,  #1396, #2288 ) ;
#1931=VERTEX_POINT ( 'NONE', #128 ) ;
#1934=CARTESIAN_POINT ( 'NONE',  ( -57.33076211353320417, -39.99999999999994316, 3.000000000000001332 ) ) ;
#1937=DIRECTION ( 'NONE',  ( -0.000000000000000000, -0.000000000000000000, -1.000000000000000000 ) ) ;
#1938=VECTOR ( 'NONE', #2868, 1000.000000000000000 ) ;
#1953=( LENGTH_UNIT ( ) NAMED_UNIT ( * ) SI_UNIT ( .MILLI., .METRE. ) );
#1960=PLANE ( 'NONE',  #1020 ) ;
#1966=CYLINDRICAL_SURFACE ( 'NONE', #2335, 2.649999999999985700 ) ;
#1968=AXIS2_PLACEMENT_3D ( 'NONE', #387, #440, #2026 ) ;
#1969=DIRECTION ( 'NONE',  ( 0.5000000000000013323, -0.8660254037844379305, 0.000000000000000000 ) ) ;
#1970=ORIENTED_EDGE ( 'NONE', *, *, #2314, .F. ) ;
#1971=AXIS2_PLACEMENT_3D ( 'NONE', #591, #2674, #623 ) ;
#1975=EDGE_LOOP ( 'NONE', ( #125, #563 ) ) ;
#1980=CARTESIAN_POINT ( 'NONE',  ( -64.98076211353318854, 10.00000000000005684, 3.000000000000000000 ) ) ;
#1981=AXIS2_PLACEMENT_3D ( 'NONE', #252, #2231, #1335 ) ;
#1983=( GEOMETRIC_REPRESENTATION_CONTEXT ( 3 ) GLOBAL_UNCERTAINTY_ASSIGNED_CONTEXT ( ( #2019 ) ) GLOBAL_UNIT_ASSIGNED_CONTEXT ( ( #1599, #266, #1225 ) ) REPRESENTATION_CONTEXT ( 'NONE', 'WORKASPACE' ) );
#1999=ORIENTED_EDGE ( 'NONE', *, *, #782, .T. ) ;
#2008=LINE ( 'NONE', #2279, #212 ) ;
#2009=CARTESIAN_POINT ( 'NONE',  ( -57.33076211353321128, -9.999999999999943157, -3.000000000000005329 ) ) ;
#2011=CARTESIAN_POINT ( 'NONE',  ( -64.98076211353316012, -131.3397459621555754, 3.000000000000000000 ) ) ;
#2017=DIRECTION ( 'NONE',  ( -0.000000000000000000, -0.000000000000000000, 1.000000000000000000 ) ) ;
#2019=UNCERTAINTY_MEASURE_WITH_UNIT (LENGTH_MEASURE( 1.000000000000000082E-05 ), #1599, 'distance_accuracy_value', 'NONE');
#2021=ORIENTED_EDGE ( 'NONE', *, *, #634, .F. ) ;
#2023=EDGE_LOOP ( 'NONE', ( #2359, #1639, #1146, #2794 ) ) ;
#2026=DIRECTION ( 'NONE',  ( 1.000000000000000000, 0.000000000000000000, 0.000000000000000000 ) ) ;
#2031=DIRECTION ( 'NONE',  ( 0.000000000000000000, 0.000000000000000000, 1.000000000000000000 ) ) ;
#2033=ORIENTED_EDGE ( 'NONE', *, *, #2782, .T. ) ;
#2038=EDGE_CURVE ( 'NONE', #1547, #2489, #2800, .T. ) ;
#2042=DIRECTION ( 'NONE',  ( -0.3420201433256743195, 0.9396926207859063185, 0.000000000000000000 ) ) ;
#2044=CIRCLE ( 'NONE', #851, 2.649999999999985700 ) ;
#2056=EDGE_CURVE ( 'NONE', #300, #741, #2595, .T. ) ;
#2061=ORIENTED_EDGE ( 'NONE', *, *, #2156, .T. ) ;
#2062=FACE_OUTER_BOUND ( 'NONE', #1732, .T. ) ;
#2068=DIRECTION ( 'NONE',  ( -1.000000000000000000, 0.000000000000000000, -0.000000000000000000 ) ) ;
#2070=VERTEX_POINT ( 'NONE', #2400 ) ;
#2078=DIRECTION ( 'NONE',  ( -0.000000000000000000, -0.000000000000000000, -1.000000000000000000 ) ) ;
#2081=AXIS2_PLACEMENT_3D ( 'NONE', #1790, #2685, #2232 ) ;
#2087=FACE_BOUND ( 'NONE', #1306, .T. ) ;
#2097=DIRECTION ( 'NONE',  ( 0.000000000000000000, 1.000000000000000000, 0.000000000000000000 ) ) ;
#2104=CARTESIAN_POINT ( 'NONE',  ( -59.98076211353319565, -9.999999999999943157, -3.000000000000005329 ) ) ;
#2110=EDGE_CURVE ( 'NONE', #1742, #741, #1291, .T. ) ;
#2116=DIRECTION ( 'NONE',  ( 1.486905836551548832E-16, -1.000000000000000000, 0.000000000000000000 ) ) ;
#2119=VECTOR ( 'NONE', #2605, 1000.000000000000000 ) ;
#2120=ORIENTED_EDGE ( 'NONE', *, *, #111, .F. ) ;
#2122=AXIS2_PLACEMENT_3D ( 'NONE', #2491, #245, #1127 ) ;
#2127=CIRCLE ( 'NONE', #1263, 2.649999999999985700 ) ;
#2128=ORIENTED_EDGE ( 'NONE', *, *, #1493, .F. ) ;
#2132=ORIENTED_EDGE ( 'NONE', *, *, #199, .F. ) ;
#2133=DIRECTION ( 'NONE',  ( 0.000000000000000000, 0.000000000000000000, -1.000000000000000000 ) ) ;
#2141=VECTOR ( 'NONE', #1685, 1000.000000000000000 ) ;
#2150=DIRECTION ( 'NONE',  ( -0.000000000000000000, -0.000000000000000000, 1.000000000000000000 ) ) ;
#2156=EDGE_CURVE ( 'NONE', #2489, #1547, #2212, .T. ) ;
#2172=AXIS2_PLACEMENT_3D ( 'NONE', #2887, #131, #2647 ) ;
#2185=FILL_AREA_STYLE ('',( #1272 ) ) ;
#2192=ADVANCED_FACE ( 'NONE', ( #1278 ), #1960, .F. ) ;
#2201=VERTEX_POINT ( 'NONE', #1857 ) ;
#2202=DIRECTION ( 'NONE',  ( -0.000000000000000000, -0.000000000000000000, -1.000000000000000000 ) ) ;
#2212=CIRCLE ( 'NONE', #1968, 2.649999999999985700 ) ;
#2213=CARTESIAN_POINT ( 'NONE',  ( -37.91455138073065001, -142.8479302707733041, 3.000000000000000000 ) ) ;
#2214=ORIENTED_EDGE ( 'NONE', *, *, #113, .T. ) ;
#2221=PRODUCT_CONTEXT ( 'NONE', #1482, 'mechanical' ) ;
#2228=DIRECTION ( 'NONE',  ( -0.000000000000000000, -0.000000000000000000, 1.000000000000000000 ) ) ;
#2230=LINE ( 'NONE', #1772, #2671 ) ;
#2231=DIRECTION ( 'NONE',  ( 0.000000000000000000, 0.000000000000000000, -1.000000000000000000 ) ) ;
#2232=DIRECTION ( 'NONE',  ( 1.000000000000000000, 0.000000000000000000, 0.000000000000000000 ) ) ;
#2236=CARTESIAN_POINT ( 'NONE',  ( -55.65063509461099045, -127.4999999999999432, 3.000000000000000000 ) ) ;
#2238=CARTESIAN_POINT ( 'NONE',  ( -64.98076211353318854, 10.00000000000005684, -3.000000000000000000 ) ) ;
#2240=VERTEX_POINT ( 'NONE', #1189 ) ;
#2243=DIRECTION ( 'NONE',  ( 1.000000000000000000, 0.000000000000000000, 0.000000000000000000 ) ) ;
#2244=CYLINDRICAL_SURFACE ( 'NONE', #792, 2.649999999999985700 ) ;
#2249=FACE_OUTER_BOUND ( 'NONE', #2709, .T. ) ;
#2255=ORIENTED_EDGE ( 'NONE', *, *, #1266, .F. ) ;
#2264=DIRECTION ( 'NONE',  ( -1.486905836551548586E-16, 1.000000000000000000, 0.000000000000000000 ) ) ;
#2273=ORIENTED_EDGE ( 'NONE', *, *, #964, .F. ) ;
#2279=CARTESIAN_POINT ( 'NONE',  ( -55.65063509461099045, -127.4999999999999432, -3.000000000000000000 ) ) ;
#2284=FACE_BOUND ( 'NONE', #1975, .T. ) ;
#2288=ADVANCED_BREP_SHAPE_REPRESENTATION ( '', ( #1538, #2652 ), #986 ) ;
#2289=ADVANCED_FACE ( 'NONE', ( #1355, #728, #716, #682 ), #2506, .T. ) ;
#2290=EDGE_LOOP ( 'NONE', ( #1014, #837 ) ) ;
#2291=FACE_OUTER_BOUND ( 'NONE', #2429, .T. ) ;
#2300=ORIENTED_EDGE ( 'NONE', *, *, #75, .T. ) ;
#2301=ORIENTED_EDGE ( 'NONE', *, *, #152, .F. ) ;
#2303=ORIENTED_EDGE ( 'NONE', *, *, #2110, .F. ) ;
#2306=DIRECTION ( 'NONE',  ( 1.486905836551548832E-16, -1.000000000000000000, 0.000000000000000000 ) ) ;
#2311=ORIENTED_EDGE ( 'NONE', *, *, #1342, .T. ) ;
#2313=ADVANCED_FACE ( 'NONE', ( #1636, #2087, #2284, #956 ), #1619, .F. ) ;
#2314=EDGE_CURVE ( 'NONE', #83, #1384, #2889, .T. ) ;
#2315=VERTEX_POINT ( 'NONE', #1869 ) ;
#2316=CIRCLE ( 'NONE', #416, 2.649999999999985700 ) ;
#2319=DIRECTION ( 'NONE',  ( -0.000000000000000000, -0.000000000000000000, -1.000000000000000000 ) ) ;
#2325=ADVANCED_FACE ( 'NONE', ( #2798 ), #1574, .T. ) ;
#2335=AXIS2_PLACEMENT_3D ( 'NONE', #2621, #1634, #2243 ) ;
#2340=CARTESIAN_POINT ( 'NONE',  ( -54.98076211353320275, 10.00000000000005684, -3.000000000000000000 ) ) ;
#2350=APPLICATION_CONTEXT ( 'automotive_design' ) ;
#2359=ORIENTED_EDGE ( 'NONE', *, *, #1622, .T. ) ;
#2360=CARTESIAN_POINT ( 'NONE',  ( -54.98076211353318143, -128.6602540378443393, -3.000000000000000000 ) ) ;
#2362=VECTOR ( 'NONE', #959, 1000.000000000000000 ) ;
#2363=EDGE_LOOP ( 'NONE', ( #1091, #2311, #487, #2416, #1710, #2120, #378, #2733, #1105 ) ) ;
#2400=CARTESIAN_POINT ( 'NONE',  ( -58.09974666316956160, -143.2580143298517328, 3.000000000000000000 ) ) ;
#2407=DIRECTION ( 'NONE',  ( -0.5000000000000013323, 0.8660254037844378194, 0.000000000000000000 ) ) ;
#2412=DIRECTION ( 'NONE',  ( 0.5000000000000013323, -0.8660254037844379305, 0.000000000000000000 ) ) ;
#2416=ORIENTED_EDGE ( 'NONE', *, *, #219, .F. ) ;
#2422=AXIS2_PLACEMENT_3D ( 'NONE', #1253, #2650, #1480 ) ;
#2429=EDGE_LOOP ( 'NONE', ( #2255, #560, #177, #2736 ) ) ;
#2430=CARTESIAN_POINT ( 'NONE',  ( -49.19086283016151384, -146.9521719906813928, 3.000000000000000000 ) ) ;
#2431=( NAMED_UNIT ( * ) SI_UNIT ( $, .STERADIAN. ) SOLID_ANGLE_UNIT ( ) );
#2438=CARTESIAN_POINT ( 'NONE',  ( -45.24838417255416800, -145.5172271100825299, 3.000000000000000000 ) ) ;
#2445=( LENGTH_UNIT ( ) NAMED_UNIT ( * ) SI_UNIT ( .MILLI., .METRE. ) );
#2453=DIRECTION ( 'NONE',  ( 1.000000000000000000, 0.000000000000000000, 0.000000000000000000 ) ) ;
#2456=VECTOR ( 'NONE', #2306, 1000.000000000000000 ) ;
#2463=CIRCLE ( 'NONE', #2081, 2.649999999999985700 ) ;
#2476=AXIS2_PLACEMENT_3D ( 'NONE', #308, #1627, #1430 ) ;
#2489=VERTEX_POINT ( 'NONE', #384 ) ;
#2491=CARTESIAN_POINT ( 'NONE',  ( -45.80724301738815285, -144.1538470861320604, 3.000000000000000000 ) ) ;
#2497=CARTESIAN_POINT ( 'NONE',  ( -49.15924597065973956, -151.4177355903189550, -3.000000000000000000 ) ) ;
#2506=PLANE ( 'NONE',  #94 ) ;
#2514=EDGE_CURVE ( 'NONE', #2201, #1508, #1496, .T. ) ;
#2515=DIRECTION ( 'NONE',  ( 1.000000000000000000, 0.000000000000000000, 0.000000000000000000 ) ) ;
#2516=EDGE_CURVE ( 'NONE', #2315, #120, #214, .T. ) ;
#2522=PLANE ( 'NONE',  #1082 ) ;
#2525=DIRECTION ( 'NONE',  ( -1.000000000000000000, 0.000000000000000000, -0.000000000000000000 ) ) ;
#2529=VERTEX_POINT ( 'NONE', #2009 ) ;
#2538=CARTESIAN_POINT ( 'NONE',  ( -59.98076211353319565, -9.999999999999943157, 3.000000000000001332 ) ) ;
#2543=DIRECTION ( 'NONE',  ( 1.486905836551548832E-16, -1.000000000000000000, 0.000000000000000000 ) ) ;
#2548=CYLINDRICAL_SURFACE ( 'NONE', #1746, 8.000000000000000000 ) ;
#2553=VECTOR ( 'NONE', #1096, 1000.000000000000000 ) ;
#2564=ORIENTED_EDGE ( 'NONE', *, *, #2682, .T. ) ;
#2566=ADVANCED_FACE ( 'NONE', ( #2917 ), #1748, .T. ) ;
#2572=DIRECTION ( 'NONE',  ( 1.000000000000000000, 0.000000000000000000, 0.000000000000000000 ) ) ;
#2574=EDGE_CURVE ( 'NONE', #2820, #1058, #2316, .T. ) ;
#2586=LINE ( 'NONE', #1893, #854 ) ;
#2595=LINE ( 'NONE', #1013, #736 ) ;
#2597=ORIENTED_EDGE ( 'NONE', *, *, #1009, .F. ) ;
#2604=CARTESIAN_POINT ( 'NONE',  ( -49.15924597065973956, -151.4177355903189550, 3.000000000000000000 ) ) ;
#2605=DIRECTION ( 'NONE',  ( 1.486905836551548832E-16, -1.000000000000000000, 0.000000000000000000 ) ) ;
#2611=CARTESIAN_POINT ( 'NONE',  ( -45.80724301738815285, -144.1538470861320604, -3.000000000000000000 ) ) ;
#2621=CARTESIAN_POINT ( 'NONE',  ( -59.98076211353318854, -69.99999999999995737, 3.000000000000000000 ) ) ;
#2628=LINE ( 'NONE', #1474, #2663 ) ;
#2633=CARTESIAN_POINT ( 'NONE',  ( -57.33076211353320417, -39.99999999999994316, 3.000000000000000000 ) ) ;
#2635=CARTESIAN_POINT ( 'NONE',  ( -64.31088913245535821, -132.4999999999999432, 3.000000000000000000 ) ) ;
#2641=LINE ( 'NONE', #2236, #1938 ) ;
#2647=DIRECTION ( 'NONE',  ( 1.000000000000000000, 0.000000000000000000, 0.000000000000000000 ) ) ;
#2650=DIRECTION ( 'NONE',  ( -0.000000000000000000, -0.000000000000000000, 1.000000000000000000 ) ) ;
#2652=AXIS2_PLACEMENT_3D ( 'NONE', #231, #2031, #1309 ) ;
#2656=MECHANICAL_DESIGN_GEOMETRIC_PRESENTATION_REPRESENTATION('',(#1691),#1924);
#2663=VECTOR ( 'NONE', #2116, 1000.000000000000000 ) ;
#2671=VECTOR ( 'NONE', #1364, 1000.000000000000000 ) ;
#2674=DIRECTION ( 'NONE',  ( 0.000000000000000000, 0.000000000000000000, -1.000000000000000000 ) ) ;
#2677=DIRECTION ( 'NONE',  ( 1.000000000000000000, 1.486905836551548586E-16, -0.000000000000000000 ) ) ;
#2681=ORIENTED_EDGE ( 'NONE', *, *, #2514, .T. ) ;
#2682=EDGE_CURVE ( 'NONE', #1508, #93, #78, .T. ) ;
#2685=DIRECTION ( 'NONE',  ( -0.000000000000000000, -0.000000000000000000, 1.000000000000000000 ) ) ;
#2698=DIRECTION ( 'NONE',  ( -0.000000000000000000, -0.000000000000000000, 1.000000000000000000 ) ) ;
#2705=ORIENTED_EDGE ( 'NONE', *, *, #129, .F. ) ;
#2709=EDGE_LOOP ( 'NONE', ( #954, #1405, #2888, #2922 ) ) ;
#2710=CIRCLE ( 'NONE', #1835, 2.649999999999985700 ) ;
#2713=DIRECTION ( 'NONE',  ( -0.000000000000000000, -0.000000000000000000, 1.000000000000000000 ) ) ;
#2720=FACE_OUTER_BOUND ( 'NONE', #1080, .T. ) ;
#2724=DIRECTION ( 'NONE',  ( -0.000000000000000000, -0.000000000000000000, 1.000000000000000000 ) ) ;
#2730=FACE_OUTER_BOUND ( 'NONE', #305, .T. ) ;
#2733=ORIENTED_EDGE ( 'NONE', *, *, #964, .T. ) ;
#2736=ORIENTED_EDGE ( 'NONE', *, *, #2574, .T. ) ;
#2737=LINE ( 'NONE', #501, #2362 ) ;
#2740=UNCERTAINTY_MEASURE_WITH_UNIT (LENGTH_MEASURE( 1.000000000000000082E-05 ), #2445, 'distance_accuracy_value', 'NONE');
#2741=DIRECTION ( 'NONE',  ( -0.000000000000000000, -0.000000000000000000, 1.000000000000000000 ) ) ;
#2745=ORIENTED_EDGE ( 'NONE', *, *, #2516, .T. ) ;
#2751=VECTOR ( 'NONE', #2078, 1000.000000000000000 ) ;
#2753=PRESENTATION_STYLE_ASSIGNMENT (( #263 ) ) ;
#2758=LINE ( 'NONE', #311, #197 ) ;
#2780=ORIENTED_EDGE ( 'NONE', *, *, #495, .F. ) ;
#2782=EDGE_CURVE ( 'NONE', #1384, #83, #788, .T. ) ;
#2792=EDGE_CURVE ( 'NONE', #1630, #2820, #1478, .T. ) ;
#2794=ORIENTED_EDGE ( 'NONE', *, *, #2056, .T. ) ;
#2797=ADVANCED_FACE ( 'NONE', ( #794 ), #1916, .F. ) ;
#2798=FACE_OUTER_BOUND ( 'NONE', #1417, .T. ) ;
#2800=CIRCLE ( 'NONE', #1822, 2.649999999999985700 ) ;
#2804=ORIENTED_EDGE ( 'NONE', *, *, #2782, .F. ) ;
#2820=VERTEX_POINT ( 'NONE', #1934 ) ;
#2834=VERTEX_POINT ( 'NONE', #390 ) ;
#2852=CARTESIAN_POINT ( 'NONE',  ( -37.80724301738815285, -144.1538470861320604, 3.000000000000000000 ) ) ;
#2867=ORIENTED_EDGE ( 'NONE', *, *, #1472, .T. ) ;
#2868=DIRECTION ( 'NONE',  ( 0.5000000000000013323, -0.8660254037844379305, 0.000000000000000000 ) ) ;
#2870=DIRECTION ( 'NONE',  ( -0.000000000000000000, -0.000000000000000000, 1.000000000000000000 ) ) ;
#2875=ORIENTED_EDGE ( 'NONE', *, *, #1472, .F. ) ;
#2887=CARTESIAN_POINT ( 'NONE',  ( -59.98076211353318854, -39.99999999999994316, 3.000000000000000000 ) ) ;
#2888=ORIENTED_EDGE ( 'NONE', *, *, #219, .T. ) ;
#2889=CIRCLE ( 'NONE', #510, 2.649999999999985700 ) ;
#2894=DIRECTION ( 'NONE',  ( -0.000000000000000000, -0.000000000000000000, -1.000000000000000000 ) ) ;
#2903=VECTOR ( 'NONE', #1927, 1000.000000000000000 ) ;
#2909=AXIS2_PLACEMENT_3D ( 'NONE', #417, #645, #223 ) ;
#2912=ORIENTED_EDGE ( 'NONE', *, *, #1428, .F. ) ;
#2915=EDGE_CURVE ( 'NONE', #908, #2070, #857, .T. ) ;
#2917=FACE_OUTER_BOUND ( 'NONE', #1341, .T. ) ;
#2922=ORIENTED_EDGE ( 'NONE', *, *, #495, .T. ) ;
#2931=ORIENTED_EDGE ( 'NONE', *, *, #1193, .T. ) ;
#2950=COLOUR_RGB('Sky Blue',0.24,0.69,0.87);
#2951=FILL_AREA_STYLE_COLOUR('',#2950);
#2952=FILL_AREA_STYLE('',(#2951));
#2953=SURFACE_STYLE_FILL_AREA(#2952);
#2954=SURFACE_SIDE_STYLE('',(#2953));
#2955=SURFACE_STYLE_USAGE(.BOTH.,#2954);
#2956=PRESENTATION_STYLE_ASSIGNMENT((#2955));
ENDSEC;
END-ISO-10303-21;
